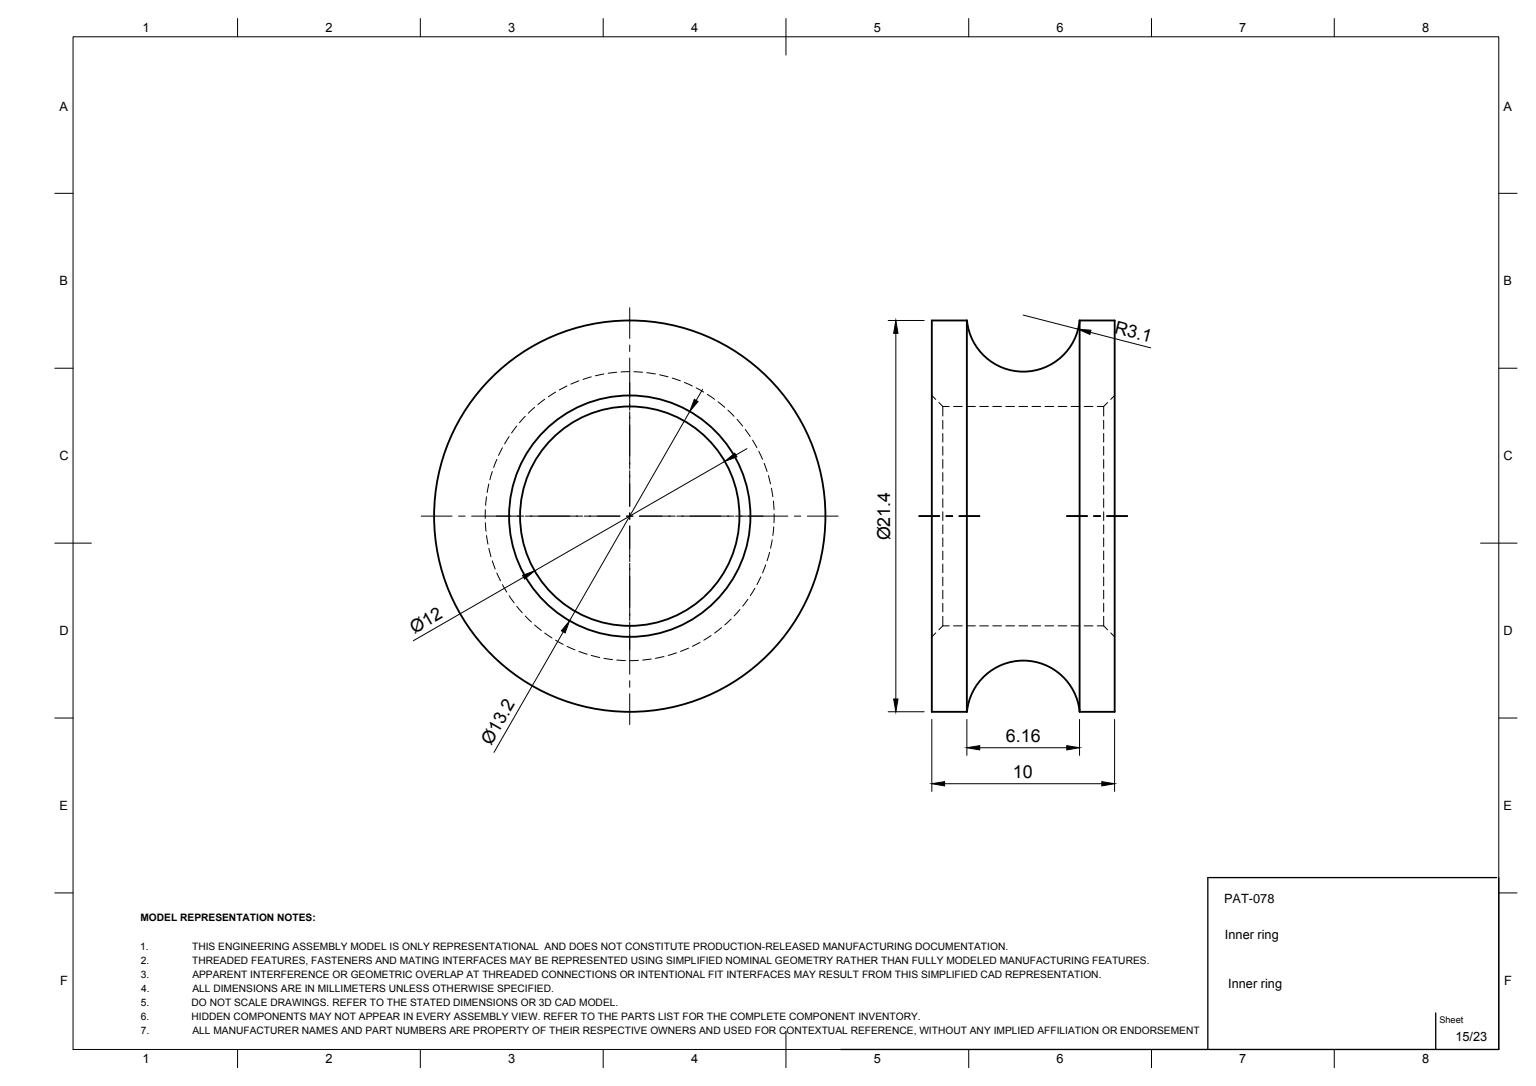
ISO-10303-21;
HEADER;
/* Generated by software containing ST-Developer
 * from STEP Tools, Inc. (www.steptools.com) 
 */

FILE_DESCRIPTION(
/* description */ ('Pedal-braked fixed caster'),
/* implementation_level */ '2;1');

FILE_NAME(
/* name */ 'Inner ring.step',
/* time_stamp */ '2026-10-28T03:26:52-07:00',
/* author */ (''),
/* organization */ (''),
/* preprocessor_version */ 'ST-DEVELOPER v20.2',
/* originating_system */ 'Autodesk Translation Framework v15.17.0.0',
/* authorisation */ '');

FILE_SCHEMA (('AUTOMOTIVE_DESIGN { 1 0 10303 214 3 1 1 }'));
ENDSEC;

DATA;
#10=MECHANICAL_DESIGN_GEOMETRIC_PRESENTATION_REPRESENTATION('',(#215),#5734);
#39=TOROIDAL_SURFACE('',#3389,1.1,0.309556);
#166=CONICAL_SURFACE('',#3400,0.63,0.785398163397448);
#167=CONICAL_SURFACE('',#3407,0.63,0.785398163397448);
#181=SHAPE_REPRESENTATION_RELATIONSHIP('SRR','None',#5821,#198);
#198=ADVANCED_BREP_SHAPE_REPRESENTATION('',(#238),#5725);
#215=STYLED_ITEM('',(#5984),#238);
#238=MANIFOLD_SOLID_BREP('Body1',#2997);
#278=CYLINDRICAL_SURFACE('',#3395,1.070235);
#279=CYLINDRICAL_SURFACE('',#3397,0.6);
#280=CYLINDRICAL_SURFACE('',#3403,1.070235);
#327=FACE_BOUND('',#799,.T.);
#328=FACE_BOUND('',#802,.T.);
#397=CIRCLE('',#3390,1.070235);
#398=CIRCLE('',#3391,1.070235);
#399=CIRCLE('',#3392,0.309556);
#400=CIRCLE('',#3393,1.070235);
#401=CIRCLE('',#3394,1.070235);
#402=CIRCLE('',#3396,1.070235);
#403=CIRCLE('',#3398,0.6);
#404=CIRCLE('',#3399,0.6);
#405=CIRCLE('',#3401,0.66);
#406=CIRCLE('',#3404,1.070235);
#407=CIRCLE('',#3406,0.66);
#584=FACE_OUTER_BOUND('',#794,.T.);
#585=FACE_OUTER_BOUND('',#795,.T.);
#586=FACE_OUTER_BOUND('',#796,.T.);
#587=FACE_OUTER_BOUND('',#797,.T.);
#588=FACE_OUTER_BOUND('',#798,.T.);
#589=FACE_OUTER_BOUND('',#800,.T.);
#590=FACE_OUTER_BOUND('',#801,.T.);
#591=FACE_OUTER_BOUND('',#803,.T.);
#794=EDGE_LOOP('',(#2406,#2407,#2408,#2409,#2410,#2411));
#795=EDGE_LOOP('',(#2412,#2413,#2414,#2415,#2416));
#796=EDGE_LOOP('',(#2417,#2418,#2419,#2420));
#797=EDGE_LOOP('',(#2421,#2422,#2423,#2424));
#798=EDGE_LOOP('',(#2425));
#799=EDGE_LOOP('',(#2426));
#800=EDGE_LOOP('',(#2427,#2428,#2429,#2430,#2431));
#801=EDGE_LOOP('',(#2432));
#802=EDGE_LOOP('',(#2433));
#803=EDGE_LOOP('',(#2434,#2435,#2436,#2437));
#1035=LINE('',#5061,#1247);
#1036=LINE('',#5067,#1248);
#1037=LINE('',#5071,#1249);
#1038=LINE('',#5077,#1250);
#1039=LINE('',#5082,#1251);
#1247=VECTOR('',#4111,1.070235);
#1248=VECTOR('',#4118,0.6);
#1249=VECTOR('',#4123,0.63);
#1250=VECTOR('',#4132,1.070235);
#1251=VECTOR('',#4139,0.63);
#1454=VERTEX_POINT('',#5050);
#1455=VERTEX_POINT('',#5051);
#1456=VERTEX_POINT('',#5054);
#1457=VERTEX_POINT('',#5056);
#1458=VERTEX_POINT('',#5060);
#1459=VERTEX_POINT('',#5064);
#1460=VERTEX_POINT('',#5066);
#1461=VERTEX_POINT('',#5070);
#1462=VERTEX_POINT('',#5075);
#1463=VERTEX_POINT('',#5079);
#1793=EDGE_CURVE('',#1454,#1455,#397,.T.);
#1794=EDGE_CURVE('',#1455,#1454,#398,.T.);
#1795=EDGE_CURVE('',#1455,#1456,#399,.T.);
#1796=EDGE_CURVE('',#1457,#1456,#400,.T.);
#1797=EDGE_CURVE('',#1456,#1457,#401,.T.);
#1798=EDGE_CURVE('',#1457,#1458,#1035,.T.);
#1799=EDGE_CURVE('',#1458,#1458,#402,.T.);
#1800=EDGE_CURVE('',#1459,#1459,#403,.T.);
#1801=EDGE_CURVE('',#1459,#1460,#1036,.T.);
#1802=EDGE_CURVE('',#1460,#1460,#404,.T.);
#1803=EDGE_CURVE('',#1460,#1461,#1037,.T.);
#1804=EDGE_CURVE('',#1461,#1461,#405,.T.);
#1805=EDGE_CURVE('',#1462,#1462,#406,.T.);
#1806=EDGE_CURVE('',#1462,#1454,#1038,.T.);
#1807=EDGE_CURVE('',#1463,#1463,#407,.T.);
#1808=EDGE_CURVE('',#1463,#1459,#1039,.T.);
#2406=ORIENTED_EDGE('',*,*,#1793,.F.);
#2407=ORIENTED_EDGE('',*,*,#1794,.F.);
#2408=ORIENTED_EDGE('',*,*,#1795,.T.);
#2409=ORIENTED_EDGE('',*,*,#1796,.F.);
#2410=ORIENTED_EDGE('',*,*,#1797,.F.);
#2411=ORIENTED_EDGE('',*,*,#1795,.F.);
#2412=ORIENTED_EDGE('',*,*,#1796,.T.);
#2413=ORIENTED_EDGE('',*,*,#1797,.T.);
#2414=ORIENTED_EDGE('',*,*,#1798,.T.);
#2415=ORIENTED_EDGE('',*,*,#1799,.T.);
#2416=ORIENTED_EDGE('',*,*,#1798,.F.);
#2417=ORIENTED_EDGE('',*,*,#1800,.T.);
#2418=ORIENTED_EDGE('',*,*,#1801,.T.);
#2419=ORIENTED_EDGE('',*,*,#1802,.F.);
#2420=ORIENTED_EDGE('',*,*,#1801,.F.);
#2421=ORIENTED_EDGE('',*,*,#1802,.T.);
#2422=ORIENTED_EDGE('',*,*,#1803,.T.);
#2423=ORIENTED_EDGE('',*,*,#1804,.F.);
#2424=ORIENTED_EDGE('',*,*,#1803,.F.);
#2425=ORIENTED_EDGE('',*,*,#1799,.F.);
#2426=ORIENTED_EDGE('',*,*,#1804,.T.);
#2427=ORIENTED_EDGE('',*,*,#1805,.F.);
#2428=ORIENTED_EDGE('',*,*,#1806,.T.);
#2429=ORIENTED_EDGE('',*,*,#1793,.T.);
#2430=ORIENTED_EDGE('',*,*,#1794,.T.);
#2431=ORIENTED_EDGE('',*,*,#1806,.F.);
#2432=ORIENTED_EDGE('',*,*,#1805,.T.);
#2433=ORIENTED_EDGE('',*,*,#1807,.F.);
#2434=ORIENTED_EDGE('',*,*,#1807,.T.);
#2435=ORIENTED_EDGE('',*,*,#1808,.T.);
#2436=ORIENTED_EDGE('',*,*,#1800,.F.);
#2437=ORIENTED_EDGE('',*,*,#1808,.F.);
#2776=PLANE('',#3402);
#2777=PLANE('',#3405);
#2917=ADVANCED_FACE('',(#584),#39,.F.);
#2918=ADVANCED_FACE('',(#585),#278,.T.);
#2919=ADVANCED_FACE('',(#586),#279,.F.);
#2920=ADVANCED_FACE('',(#587),#166,.F.);
#2921=ADVANCED_FACE('',(#588,#327),#2776,.T.);
#2922=ADVANCED_FACE('',(#589),#280,.T.);
#2923=ADVANCED_FACE('',(#590,#328),#2777,.T.);
#2924=ADVANCED_FACE('',(#591),#167,.F.);
#2997=CLOSED_SHELL('',(#2917,#2918,#2919,#2920,#2921,#2922,#2923,#2924));
#3388=AXIS2_PLACEMENT_3D('',#5048,#4095,#4096);
#3389=AXIS2_PLACEMENT_3D('',#5049,#4097,#4098);
#3390=AXIS2_PLACEMENT_3D('',#5052,#4099,#4100);
#3391=AXIS2_PLACEMENT_3D('',#5053,#4101,#4102);
#3392=AXIS2_PLACEMENT_3D('',#5055,#4103,#4104);
#3393=AXIS2_PLACEMENT_3D('',#5057,#4105,#4106);
#3394=AXIS2_PLACEMENT_3D('',#5058,#4107,#4108);
#3395=AXIS2_PLACEMENT_3D('',#5059,#4109,#4110);
#3396=AXIS2_PLACEMENT_3D('',#5062,#4112,#4113);
#3397=AXIS2_PLACEMENT_3D('',#5063,#4114,#4115);
#3398=AXIS2_PLACEMENT_3D('',#5065,#4116,#4117);
#3399=AXIS2_PLACEMENT_3D('',#5068,#4119,#4120);
#3400=AXIS2_PLACEMENT_3D('',#5069,#4121,#4122);
#3401=AXIS2_PLACEMENT_3D('',#5072,#4124,#4125);
#3402=AXIS2_PLACEMENT_3D('',#5073,#4126,#4127);
#3403=AXIS2_PLACEMENT_3D('',#5074,#4128,#4129);
#3404=AXIS2_PLACEMENT_3D('',#5076,#4130,#4131);
#3405=AXIS2_PLACEMENT_3D('',#5078,#4133,#4134);
#3406=AXIS2_PLACEMENT_3D('',#5080,#4135,#4136);
#3407=AXIS2_PLACEMENT_3D('',#5081,#4137,#4138);
#4095=DIRECTION('axis',(0.,0.,1.));
#4096=DIRECTION('refdir',(1.,0.,0.));
#4097=DIRECTION('center_axis',(0.,-1.,0.));
#4098=DIRECTION('ref_axis',(0.,0.,-1.));
#4099=DIRECTION('center_axis',(0.,-1.,0.));
#4100=DIRECTION('ref_axis',(1.,0.,0.));
#4101=DIRECTION('center_axis',(0.,-1.,0.));
#4102=DIRECTION('ref_axis',(1.,0.,0.));
#4103=DIRECTION('center_axis',(1.,0.,1.22464679914735E-16));
#4104=DIRECTION('ref_axis',(-1.22464679914735E-16,0.,1.));
#4105=DIRECTION('center_axis',(0.,1.,0.));
#4106=DIRECTION('ref_axis',(1.,0.,0.));
#4107=DIRECTION('center_axis',(0.,1.,0.));
#4108=DIRECTION('ref_axis',(1.,0.,0.));
#4109=DIRECTION('center_axis',(0.,-1.,0.));
#4110=DIRECTION('ref_axis',(1.,0.,0.));
#4111=DIRECTION('',(0.,1.,0.));
#4112=DIRECTION('center_axis',(0.,-1.,0.));
#4113=DIRECTION('ref_axis',(1.,0.,0.));
#4114=DIRECTION('center_axis',(0.,-1.,0.));
#4115=DIRECTION('ref_axis',(1.,0.,0.));
#4116=DIRECTION('center_axis',(0.,-1.,0.));
#4117=DIRECTION('ref_axis',(1.,0.,0.));
#4118=DIRECTION('',(0.,1.,0.));
#4119=DIRECTION('center_axis',(0.,-1.,0.));
#4120=DIRECTION('ref_axis',(1.,0.,0.));
#4121=DIRECTION('center_axis',(0.,1.,0.));
#4122=DIRECTION('ref_axis',(1.,0.,0.));
#4123=DIRECTION('',(-0.707106781186548,0.707106781186547,-8.65956056235493E-17));
#4124=DIRECTION('center_axis',(0.,-1.,0.));
#4125=DIRECTION('ref_axis',(1.,0.,0.));
#4126=DIRECTION('center_axis',(0.,1.,0.));
#4127=DIRECTION('ref_axis',(0.,0.,1.));
#4128=DIRECTION('center_axis',(0.,-1.,0.));
#4129=DIRECTION('ref_axis',(1.,0.,0.));
#4130=DIRECTION('center_axis',(0.,-1.,0.));
#4131=DIRECTION('ref_axis',(1.,0.,0.));
#4132=DIRECTION('',(0.,1.,0.));
#4133=DIRECTION('center_axis',(0.,-1.,0.));
#4134=DIRECTION('ref_axis',(0.,0.,-1.));
#4135=DIRECTION('center_axis',(0.,-1.,0.));
#4136=DIRECTION('ref_axis',(1.,0.,0.));
#4137=DIRECTION('center_axis',(0.,-1.,0.));
#4138=DIRECTION('ref_axis',(1.,0.,0.));
#4139=DIRECTION('',(0.707106781186548,0.707106781186547,8.65956056235493E-17));
#5048=CARTESIAN_POINT('',(0.,0.,0.));
#5049=CARTESIAN_POINT('Origin',(0.,0.,0.));
#5050=CARTESIAN_POINT('',(-1.070235,-0.308121667383195,-1.31065986708547E-16));
#5051=CARTESIAN_POINT('',(-1.31065986708547E-16,-0.308121667383195,1.070235));
#5052=CARTESIAN_POINT('Origin',(0.,-0.308121667383195,0.));
#5053=CARTESIAN_POINT('Origin',(0.,-0.308121667383195,0.));
#5054=CARTESIAN_POINT('',(-1.31065986708547E-16,0.308121667383195,1.070235));
#5055=CARTESIAN_POINT('Origin',(-1.34711147906209E-16,0.,1.1));
#5056=CARTESIAN_POINT('',(-1.070235,0.308121667383195,1.31065986708547E-16));
#5057=CARTESIAN_POINT('Origin',(0.,0.308121667383195,0.));
#5058=CARTESIAN_POINT('Origin',(0.,0.308121667383195,0.));
#5059=CARTESIAN_POINT('Origin',(0.,0.,0.));
#5060=CARTESIAN_POINT('',(-1.070235,0.5,-1.31065986708547E-16));
#5061=CARTESIAN_POINT('',(-1.070235,0.,-1.31065986708547E-16));
#5062=CARTESIAN_POINT('Origin',(0.,0.5,0.));
#5063=CARTESIAN_POINT('Origin',(0.,0.,0.));
#5064=CARTESIAN_POINT('',(-0.6,-0.44,-7.34788079488412E-17));
#5065=CARTESIAN_POINT('Origin',(0.,-0.44,0.));
#5066=CARTESIAN_POINT('',(-0.6,0.44,-7.34788079488412E-17));
#5067=CARTESIAN_POINT('',(-0.6,0.,-7.34788079488412E-17));
#5068=CARTESIAN_POINT('Origin',(0.,0.44,0.));
#5069=CARTESIAN_POINT('Origin',(0.,0.47,0.));
#5070=CARTESIAN_POINT('',(-0.66,0.5,-8.08266887437253E-17));
#5071=CARTESIAN_POINT('',(-0.63,0.47,-7.71527483462832E-17));
#5072=CARTESIAN_POINT('Origin',(0.,0.5,0.));
#5073=CARTESIAN_POINT('Origin',(1.070235,0.5,0.));
#5074=CARTESIAN_POINT('Origin',(0.,0.,0.));
#5075=CARTESIAN_POINT('',(-1.070235,-0.5,-1.31065986708547E-16));
#5076=CARTESIAN_POINT('Origin',(0.,-0.5,0.));
#5077=CARTESIAN_POINT('',(-1.070235,0.,-1.31065986708547E-16));
#5078=CARTESIAN_POINT('Origin',(0.66,-0.5,0.));
#5079=CARTESIAN_POINT('',(-0.66,-0.5,-8.08266887437253E-17));
#5080=CARTESIAN_POINT('Origin',(0.,-0.5,0.));
#5081=CARTESIAN_POINT('Origin',(0.,-0.47,0.));
#5082=CARTESIAN_POINT('',(-0.63,-0.47,-7.71527483462832E-17));
#5702=UNCERTAINTY_MEASURE_WITH_UNIT(LENGTH_MEASURE(0.001),#5735,
'DISTANCE_ACCURACY_VALUE',
'Maximum model space distance between geometric entities at asserted c
onnectivities');
#5711=UNCERTAINTY_MEASURE_WITH_UNIT(LENGTH_MEASURE(0.001),#5735,
'DISTANCE_ACCURACY_VALUE',
'Maximum model space distance between geometric entities at asserted c
onnectivities');
#5725=(
GEOMETRIC_REPRESENTATION_CONTEXT(3)
GLOBAL_UNCERTAINTY_ASSIGNED_CONTEXT((#5702))
GLOBAL_UNIT_ASSIGNED_CONTEXT((#5735,#5737,#5738))
REPRESENTATION_CONTEXT('','3D')
);
#5734=(
GEOMETRIC_REPRESENTATION_CONTEXT(3)
GLOBAL_UNCERTAINTY_ASSIGNED_CONTEXT((#5711))
GLOBAL_UNIT_ASSIGNED_CONTEXT((#5735,#5737,#5738))
REPRESENTATION_CONTEXT('','3D')
);
#5735=(
LENGTH_UNIT()
NAMED_UNIT(*)
SI_UNIT(.CENTI.,.METRE.)
);
#5737=(
NAMED_UNIT(*)
PLANE_ANGLE_UNIT()
SI_UNIT($,.RADIAN.)
);
#5738=(
NAMED_UNIT(*)
SI_UNIT($,.STERADIAN.)
SOLID_ANGLE_UNIT()
);
#5752=SHAPE_DEFINITION_REPRESENTATION(#5784,#5821);
#5784=PRODUCT_DEFINITION_SHAPE('',$,#5844);
#5821=SHAPE_REPRESENTATION('',(#3388),#5725);
#5830=PRODUCT_DEFINITION_CONTEXT('part definition',#5898,'design');
#5844=PRODUCT_DEFINITION('Inner ring','Inner ring',#5866,#5830);
#5866=PRODUCT_DEFINITION_FORMATION('',$,#5913);
#5898=APPLICATION_CONTEXT(
'Core Data for Automotive Mechanical Design Process');
#5899=PRODUCT_CONTEXT('part definition',#5898,'mechanical');
#5913=PRODUCT('Inner ring','Inner ring','Inner ring',(#5899));
#5978=COLOUR_RGB('Grey',0.48,0.52,0.57);
#5979=FILL_AREA_STYLE_COLOUR('',#5978);
#5980=FILL_AREA_STYLE('',(#5979));
#5981=SURFACE_STYLE_FILL_AREA(#5980);
#5982=SURFACE_SIDE_STYLE('',(#5981));
#5983=SURFACE_STYLE_USAGE(.BOTH.,#5982);
#5984=PRESENTATION_STYLE_ASSIGNMENT((#5983));
ENDSEC;
END-ISO-10303-21;
